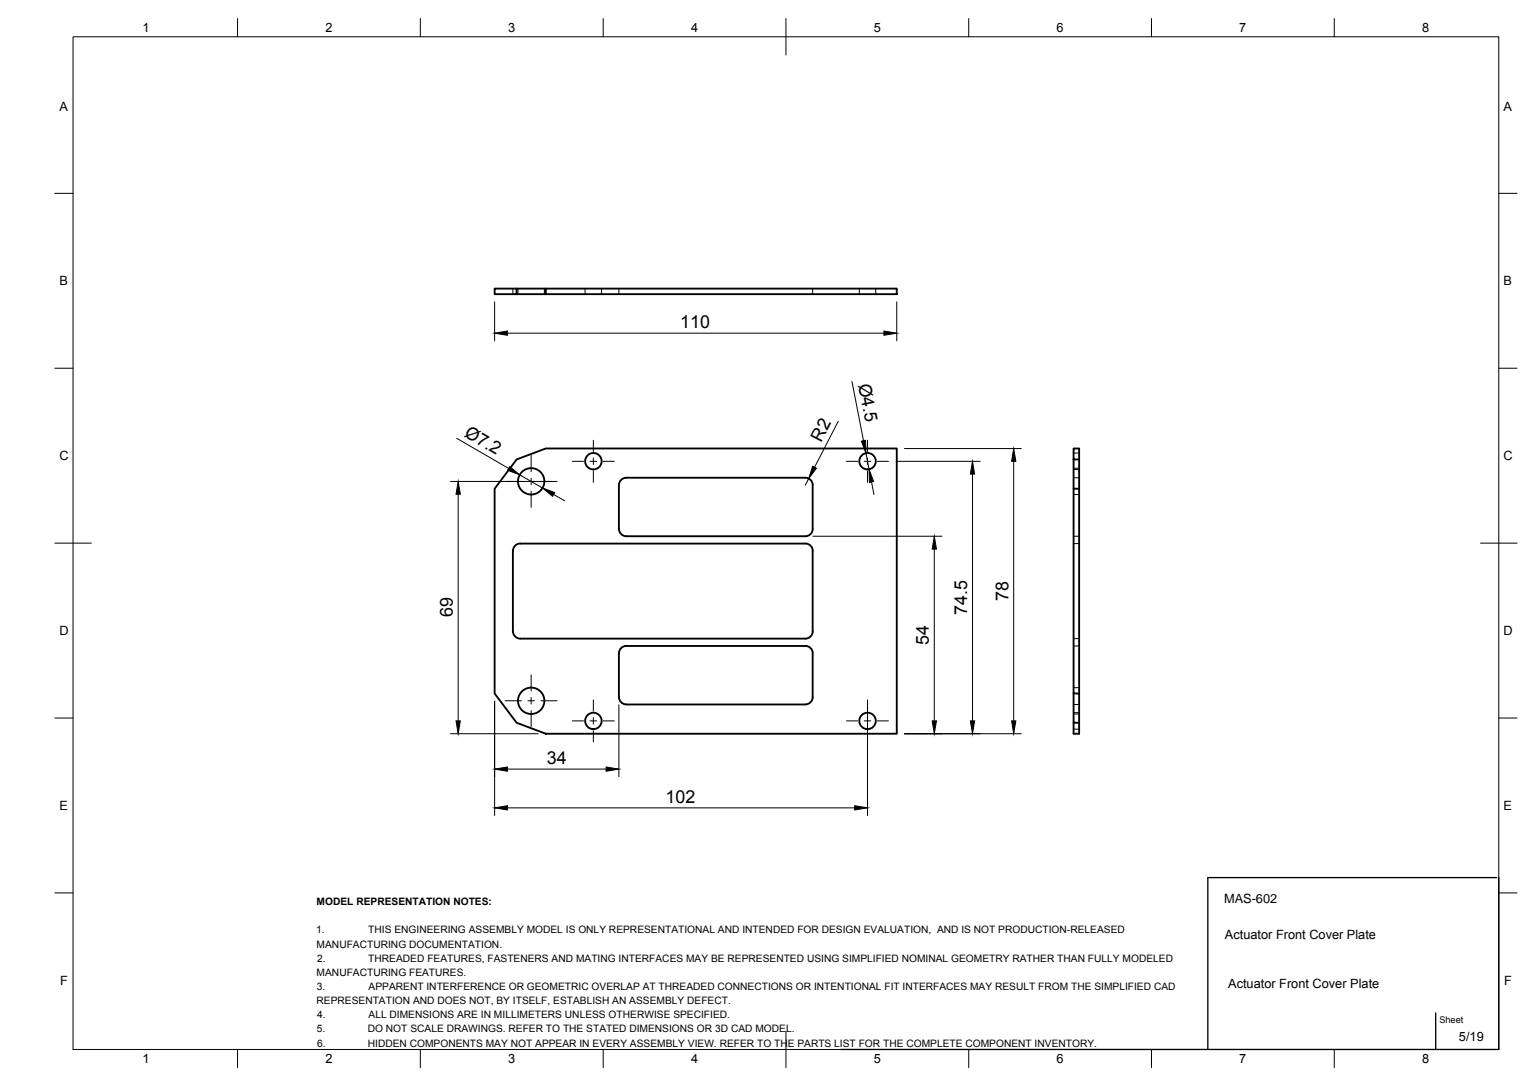
ISO-10303-21;
HEADER;
/* Generated by software containing ST-Developer
 * from STEP Tools, Inc. (www.steptools.com) 
 */

FILE_DESCRIPTION(
/* description */ (''),
/* implementation_level */ '2;1');

FILE_NAME(
/* name */ 'Actuator Front Cover Plate.step',
/* time_stamp */ '2026-10-15T14:42:47-07:00',
/* author */ (''),
/* organization */ (''),
/* preprocessor_version */ 'ST-DEVELOPER v20.2',
/* originating_system */ 'Autodesk Translation Framework v15.15.0.0',
/* authorisation */ '');

FILE_SCHEMA (('AUTOMOTIVE_DESIGN { 1 0 10303 214 3 1 1 }'));
ENDSEC;

DATA;
#10=MECHANICAL_DESIGN_GEOMETRIC_PRESENTATION_REPRESENTATION('',(#236),#85789);
#200=SHAPE_REPRESENTATION_RELATIONSHIP('SRR','None',#85865,#218);
#218=ADVANCED_BREP_SHAPE_REPRESENTATION('',(#254),#85773);
#236=STYLED_ITEM('',(#85964),#254);
#254=MANIFOLD_SOLID_BREP('Body1',#9883);
#411=FACE_BOUND('',#3173,.T.);
#412=FACE_BOUND('',#3174,.T.);
#413=FACE_BOUND('',#3175,.T.);
#414=FACE_BOUND('',#3176,.T.);
#415=FACE_BOUND('',#3177,.T.);
#416=FACE_BOUND('',#3178,.T.);
#417=FACE_BOUND('',#3179,.T.);
#418=FACE_BOUND('',#3180,.T.);
#419=FACE_BOUND('',#3181,.T.);
#420=FACE_BOUND('',#3183,.T.);
#421=FACE_BOUND('',#3184,.T.);
#422=FACE_BOUND('',#3185,.T.);
#423=FACE_BOUND('',#3186,.T.);
#424=FACE_BOUND('',#3187,.T.);
#425=FACE_BOUND('',#3188,.T.);
#426=FACE_BOUND('',#3189,.T.);
#427=FACE_BOUND('',#3190,.T.);
#428=FACE_BOUND('',#3191,.T.);
#1044=PLANE('',#10380);
#1045=PLANE('',#10384);
#1046=PLANE('',#10388);
#1047=PLANE('',#10392);
#1048=PLANE('',#10396);
#1049=PLANE('',#10400);
#1050=PLANE('',#10404);
#1051=PLANE('',#10408);
#1052=PLANE('',#10412);
#1053=PLANE('',#10416);
#1054=PLANE('',#10420);
#1055=PLANE('',#10424);
#1056=PLANE('',#10443);
#1057=PLANE('',#10444);
#1058=PLANE('',#10445);
#1059=PLANE('',#10446);
#1060=PLANE('',#10447);
#1061=PLANE('',#10448);
#1062=PLANE('',#10449);
#1063=PLANE('',#10450);
#1064=PLANE('',#10451);
#1065=PLANE('',#10452);
#1357=LINE('',#23580,#1893);
#1358=LINE('',#23583,#1894);
#1359=LINE('',#23586,#1895);
#1360=LINE('',#23588,#1896);
#1361=LINE('',#23589,#1897);
#1362=LINE('',#23595,#1898);
#1363=LINE('',#23598,#1899);
#1364=LINE('',#23600,#1900);
#1365=LINE('',#23601,#1901);
#1366=LINE('',#23606,#1902);
#1367=LINE('',#23610,#1903);
#1368=LINE('',#23612,#1904);
#1369=LINE('',#23613,#1905);
#1370=LINE('',#23618,#1906);
#1371=LINE('',#23621,#1907);
#1372=LINE('',#23622,#1908);
#1373=LINE('',#23628,#1909);
#1374=LINE('',#23631,#1910);
#1375=LINE('',#23634,#1911);
#1376=LINE('',#23636,#1912);
#1377=LINE('',#23637,#1913);
#1378=LINE('',#23643,#1914);
#1379=LINE('',#23646,#1915);
#1380=LINE('',#23648,#1916);
#1381=LINE('',#23649,#1917);
#1382=LINE('',#23654,#1918);
#1383=LINE('',#23658,#1919);
#1384=LINE('',#23660,#1920);
#1385=LINE('',#23661,#1921);
#1386=LINE('',#23666,#1922);
#1387=LINE('',#23669,#1923);
#1388=LINE('',#23670,#1924);
#1389=LINE('',#23676,#1925);
#1390=LINE('',#23679,#1926);
#1391=LINE('',#23682,#1927);
#1392=LINE('',#23684,#1928);
#1393=LINE('',#23685,#1929);
#1394=LINE('',#23691,#1930);
#1395=LINE('',#23694,#1931);
#1396=LINE('',#23696,#1932);
#1397=LINE('',#23697,#1933);
#1398=LINE('',#23702,#1934);
#1399=LINE('',#23706,#1935);
#1400=LINE('',#23708,#1936);
#1401=LINE('',#23709,#1937);
#1402=LINE('',#23714,#1938);
#1403=LINE('',#23717,#1939);
#1404=LINE('',#23718,#1940);
#1405=LINE('',#23723,#1941);
#1406=LINE('',#23729,#1942);
#1407=LINE('',#23735,#1943);
#1408=LINE('',#23741,#1944);
#1409=LINE('',#23747,#1945);
#1410=LINE('',#23753,#1946);
#1411=LINE('',#23758,#1947);
#1412=LINE('',#23760,#1948);
#1413=LINE('',#23762,#1949);
#1414=LINE('',#23763,#1950);
#1415=LINE('',#23766,#1951);
#1416=LINE('',#23768,#1952);
#1417=LINE('',#23769,#1953);
#1418=LINE('',#23772,#1954);
#1419=LINE('',#23774,#1955);
#1420=LINE('',#23775,#1956);
#1421=LINE('',#23778,#1957);
#1422=LINE('',#23780,#1958);
#1423=LINE('',#23781,#1959);
#1424=LINE('',#23784,#1960);
#1425=LINE('',#23786,#1961);
#1426=LINE('',#23787,#1962);
#1427=LINE('',#23790,#1963);
#1428=LINE('',#23792,#1964);
#1429=LINE('',#23793,#1965);
#1430=LINE('',#23796,#1966);
#1431=LINE('',#23798,#1967);
#1432=LINE('',#23799,#1968);
#1433=LINE('',#23801,#1969);
#1434=LINE('',#23802,#1970);
#1893=VECTOR('',#11679,1.);
#1894=VECTOR('',#11682,1.);
#1895=VECTOR('',#11685,1.);
#1896=VECTOR('',#11686,1.);
#1897=VECTOR('',#11687,1.);
#1898=VECTOR('',#11692,1.);
#1899=VECTOR('',#11695,1.);
#1900=VECTOR('',#11698,1.);
#1901=VECTOR('',#11699,1.);
#1902=VECTOR('',#11704,1.);
#1903=VECTOR('',#11709,1.);
#1904=VECTOR('',#11710,1.);
#1905=VECTOR('',#11711,1.);
#1906=VECTOR('',#11716,1.);
#1907=VECTOR('',#11721,1.);
#1908=VECTOR('',#11722,1.);
#1909=VECTOR('',#11727,1.);
#1910=VECTOR('',#11730,1.);
#1911=VECTOR('',#11733,1.);
#1912=VECTOR('',#11734,1.);
#1913=VECTOR('',#11735,1.);
#1914=VECTOR('',#11740,1.);
#1915=VECTOR('',#11743,1.);
#1916=VECTOR('',#11746,1.);
#1917=VECTOR('',#11747,1.);
#1918=VECTOR('',#11752,1.);
#1919=VECTOR('',#11757,1.);
#1920=VECTOR('',#11758,1.);
#1921=VECTOR('',#11759,1.);
#1922=VECTOR('',#11764,1.);
#1923=VECTOR('',#11769,1.);
#1924=VECTOR('',#11770,1.);
#1925=VECTOR('',#11775,1.);
#1926=VECTOR('',#11778,1.);
#1927=VECTOR('',#11781,1.);
#1928=VECTOR('',#11782,1.);
#1929=VECTOR('',#11783,1.);
#1930=VECTOR('',#11788,1.);
#1931=VECTOR('',#11791,1.);
#1932=VECTOR('',#11794,1.);
#1933=VECTOR('',#11795,1.);
#1934=VECTOR('',#11800,1.);
#1935=VECTOR('',#11805,1.);
#1936=VECTOR('',#11806,1.);
#1937=VECTOR('',#11807,1.);
#1938=VECTOR('',#11812,1.);
#1939=VECTOR('',#11817,1.);
#1940=VECTOR('',#11818,1.);
#1941=VECTOR('',#11823,0.225);
#1942=VECTOR('',#11830,0.36);
#1943=VECTOR('',#11837,0.36);
#1944=VECTOR('',#11844,0.225);
#1945=VECTOR('',#11851,0.225);
#1946=VECTOR('',#11858,0.225);
#1947=VECTOR('',#11863,1.);
#1948=VECTOR('',#11864,1.);
#1949=VECTOR('',#11865,1.);
#1950=VECTOR('',#11866,1.);
#1951=VECTOR('',#11869,1.);
#1952=VECTOR('',#11870,1.);
#1953=VECTOR('',#11871,1.);
#1954=VECTOR('',#11874,1.);
#1955=VECTOR('',#11875,1.);
#1956=VECTOR('',#11876,1.);
#1957=VECTOR('',#11879,1.);
#1958=VECTOR('',#11880,1.);
#1959=VECTOR('',#11881,1.);
#1960=VECTOR('',#11884,1.);
#1961=VECTOR('',#11885,1.);
#1962=VECTOR('',#11886,1.);
#1963=VECTOR('',#11889,1.);
#1964=VECTOR('',#11890,1.);
#1965=VECTOR('',#11891,1.);
#1966=VECTOR('',#11894,1.);
#1967=VECTOR('',#11895,1.);
#1968=VECTOR('',#11896,1.);
#1969=VECTOR('',#11899,1.);
#1970=VECTOR('',#11900,1.);
#2304=CYLINDRICAL_SURFACE('',#10377,0.2);
#2305=CYLINDRICAL_SURFACE('',#10381,0.2);
#2306=CYLINDRICAL_SURFACE('',#10385,0.2);
#2307=CYLINDRICAL_SURFACE('',#10389,0.2);
#2308=CYLINDRICAL_SURFACE('',#10393,0.2);
#2309=CYLINDRICAL_SURFACE('',#10397,0.2);
#2310=CYLINDRICAL_SURFACE('',#10401,0.2);
#2311=CYLINDRICAL_SURFACE('',#10405,0.2);
#2312=CYLINDRICAL_SURFACE('',#10409,0.2);
#2313=CYLINDRICAL_SURFACE('',#10413,0.2);
#2314=CYLINDRICAL_SURFACE('',#10417,0.2);
#2315=CYLINDRICAL_SURFACE('',#10421,0.2);
#2316=CYLINDRICAL_SURFACE('',#10425,0.225);
#2317=CYLINDRICAL_SURFACE('',#10428,0.36);
#2318=CYLINDRICAL_SURFACE('',#10431,0.36);
#2319=CYLINDRICAL_SURFACE('',#10434,0.225);
#2320=CYLINDRICAL_SURFACE('',#10437,0.225);
#2321=CYLINDRICAL_SURFACE('',#10440,0.225);
#2608=FACE_OUTER_BOUND('',#3134,.T.);
#2609=FACE_OUTER_BOUND('',#3135,.T.);
#2610=FACE_OUTER_BOUND('',#3136,.T.);
#2611=FACE_OUTER_BOUND('',#3137,.T.);
#2612=FACE_OUTER_BOUND('',#3138,.T.);
#2613=FACE_OUTER_BOUND('',#3139,.T.);
#2614=FACE_OUTER_BOUND('',#3140,.T.);
#2615=FACE_OUTER_BOUND('',#3141,.T.);
#2616=FACE_OUTER_BOUND('',#3142,.T.);
#2617=FACE_OUTER_BOUND('',#3143,.T.);
#2618=FACE_OUTER_BOUND('',#3144,.T.);
#2619=FACE_OUTER_BOUND('',#3145,.T.);
#2620=FACE_OUTER_BOUND('',#3146,.T.);
#2621=FACE_OUTER_BOUND('',#3147,.T.);
#2622=FACE_OUTER_BOUND('',#3148,.T.);
#2623=FACE_OUTER_BOUND('',#3149,.T.);
#2624=FACE_OUTER_BOUND('',#3150,.T.);
#2625=FACE_OUTER_BOUND('',#3151,.T.);
#2626=FACE_OUTER_BOUND('',#3152,.T.);
#2627=FACE_OUTER_BOUND('',#3153,.T.);
#2628=FACE_OUTER_BOUND('',#3154,.T.);
#2629=FACE_OUTER_BOUND('',#3155,.T.);
#2630=FACE_OUTER_BOUND('',#3156,.T.);
#2631=FACE_OUTER_BOUND('',#3157,.T.);
#2632=FACE_OUTER_BOUND('',#3158,.T.);
#2633=FACE_OUTER_BOUND('',#3159,.T.);
#2634=FACE_OUTER_BOUND('',#3160,.T.);
#2635=FACE_OUTER_BOUND('',#3161,.T.);
#2636=FACE_OUTER_BOUND('',#3162,.T.);
#2637=FACE_OUTER_BOUND('',#3163,.T.);
#2638=FACE_OUTER_BOUND('',#3164,.T.);
#2639=FACE_OUTER_BOUND('',#3165,.T.);
#2640=FACE_OUTER_BOUND('',#3166,.T.);
#2641=FACE_OUTER_BOUND('',#3167,.T.);
#2642=FACE_OUTER_BOUND('',#3168,.T.);
#2643=FACE_OUTER_BOUND('',#3169,.T.);
#2644=FACE_OUTER_BOUND('',#3170,.T.);
#2645=FACE_OUTER_BOUND('',#3171,.T.);
#2646=FACE_OUTER_BOUND('',#3172,.T.);
#2647=FACE_OUTER_BOUND('',#3182,.T.);
#3134=EDGE_LOOP('',(#7413,#7414,#7415,#7416));
#3135=EDGE_LOOP('',(#7417,#7418,#7419,#7420));
#3136=EDGE_LOOP('',(#7421,#7422,#7423,#7424));
#3137=EDGE_LOOP('',(#7425,#7426,#7427,#7428));
#3138=EDGE_LOOP('',(#7429,#7430,#7431,#7432));
#3139=EDGE_LOOP('',(#7433,#7434,#7435,#7436));
#3140=EDGE_LOOP('',(#7437,#7438,#7439,#7440));
#3141=EDGE_LOOP('',(#7441,#7442,#7443,#7444));
#3142=EDGE_LOOP('',(#7445,#7446,#7447,#7448));
#3143=EDGE_LOOP('',(#7449,#7450,#7451,#7452));
#3144=EDGE_LOOP('',(#7453,#7454,#7455,#7456));
#3145=EDGE_LOOP('',(#7457,#7458,#7459,#7460));
#3146=EDGE_LOOP('',(#7461,#7462,#7463,#7464));
#3147=EDGE_LOOP('',(#7465,#7466,#7467,#7468));
#3148=EDGE_LOOP('',(#7469,#7470,#7471,#7472));
#3149=EDGE_LOOP('',(#7473,#7474,#7475,#7476));
#3150=EDGE_LOOP('',(#7477,#7478,#7479,#7480));
#3151=EDGE_LOOP('',(#7481,#7482,#7483,#7484));
#3152=EDGE_LOOP('',(#7485,#7486,#7487,#7488));
#3153=EDGE_LOOP('',(#7489,#7490,#7491,#7492));
#3154=EDGE_LOOP('',(#7493,#7494,#7495,#7496));
#3155=EDGE_LOOP('',(#7497,#7498,#7499,#7500));
#3156=EDGE_LOOP('',(#7501,#7502,#7503,#7504));
#3157=EDGE_LOOP('',(#7505,#7506,#7507,#7508));
#3158=EDGE_LOOP('',(#7509,#7510,#7511,#7512));
#3159=EDGE_LOOP('',(#7513,#7514,#7515,#7516));
#3160=EDGE_LOOP('',(#7517,#7518,#7519,#7520));
#3161=EDGE_LOOP('',(#7521,#7522,#7523,#7524));
#3162=EDGE_LOOP('',(#7525,#7526,#7527,#7528));
#3163=EDGE_LOOP('',(#7529,#7530,#7531,#7532));
#3164=EDGE_LOOP('',(#7533,#7534,#7535,#7536));
#3165=EDGE_LOOP('',(#7537,#7538,#7539,#7540));
#3166=EDGE_LOOP('',(#7541,#7542,#7543,#7544));
#3167=EDGE_LOOP('',(#7545,#7546,#7547,#7548));
#3168=EDGE_LOOP('',(#7549,#7550,#7551,#7552));
#3169=EDGE_LOOP('',(#7553,#7554,#7555,#7556));
#3170=EDGE_LOOP('',(#7557,#7558,#7559,#7560));
#3171=EDGE_LOOP('',(#7561,#7562,#7563,#7564));
#3172=EDGE_LOOP('',(#7565,#7566,#7567,#7568,#7569,#7570,#7571,#7572));
#3173=EDGE_LOOP('',(#7573));
#3174=EDGE_LOOP('',(#7574));
#3175=EDGE_LOOP('',(#7575));
#3176=EDGE_LOOP('',(#7576));
#3177=EDGE_LOOP('',(#7577));
#3178=EDGE_LOOP('',(#7578));
#3179=EDGE_LOOP('',(#7579,#7580,#7581,#7582,#7583,#7584,#7585,#7586));
#3180=EDGE_LOOP('',(#7587,#7588,#7589,#7590,#7591,#7592,#7593,#7594));
#3181=EDGE_LOOP('',(#7595,#7596,#7597,#7598,#7599,#7600,#7601,#7602));
#3182=EDGE_LOOP('',(#7603,#7604,#7605,#7606,#7607,#7608,#7609,#7610));
#3183=EDGE_LOOP('',(#7611));
#3184=EDGE_LOOP('',(#7612));
#3185=EDGE_LOOP('',(#7613));
#3186=EDGE_LOOP('',(#7614));
#3187=EDGE_LOOP('',(#7615));
#3188=EDGE_LOOP('',(#7616));
#3189=EDGE_LOOP('',(#7617,#7618,#7619,#7620,#7621,#7622,#7623,#7624));
#3190=EDGE_LOOP('',(#7625,#7626,#7627,#7628,#7629,#7630,#7631,#7632));
#3191=EDGE_LOOP('',(#7633,#7634,#7635,#7636,#7637,#7638,#7639,#7640));
#3648=CIRCLE('',#10378,0.2);
#3649=CIRCLE('',#10379,0.2);
#3650=CIRCLE('',#10382,0.2);
#3651=CIRCLE('',#10383,0.2);
#3652=CIRCLE('',#10386,0.2);
#3653=CIRCLE('',#10387,0.2);
#3654=CIRCLE('',#10390,0.2);
#3655=CIRCLE('',#10391,0.2);
#3656=CIRCLE('',#10394,0.2);
#3657=CIRCLE('',#10395,0.2);
#3658=CIRCLE('',#10398,0.2);
#3659=CIRCLE('',#10399,0.2);
#3660=CIRCLE('',#10402,0.2);
#3661=CIRCLE('',#10403,0.2);
#3662=CIRCLE('',#10406,0.2);
#3663=CIRCLE('',#10407,0.2);
#3664=CIRCLE('',#10410,0.2);
#3665=CIRCLE('',#10411,0.2);
#3666=CIRCLE('',#10414,0.2);
#3667=CIRCLE('',#10415,0.2);
#3668=CIRCLE('',#10418,0.2);
#3669=CIRCLE('',#10419,0.2);
#3670=CIRCLE('',#10422,0.2);
#3671=CIRCLE('',#10423,0.2);
#3672=CIRCLE('',#10426,0.225);
#3673=CIRCLE('',#10427,0.225);
#3674=CIRCLE('',#10429,0.36);
#3675=CIRCLE('',#10430,0.36);
#3676=CIRCLE('',#10432,0.36);
#3677=CIRCLE('',#10433,0.36);
#3678=CIRCLE('',#10435,0.225);
#3679=CIRCLE('',#10436,0.225);
#3680=CIRCLE('',#10438,0.225);
#3681=CIRCLE('',#10439,0.225);
#3682=CIRCLE('',#10441,0.225);
#3683=CIRCLE('',#10442,0.225);
#4199=VERTEX_POINT('',#23576);
#4200=VERTEX_POINT('',#23577);
#4201=VERTEX_POINT('',#23579);
#4202=VERTEX_POINT('',#23581);
#4203=VERTEX_POINT('',#23585);
#4204=VERTEX_POINT('',#23587);
#4205=VERTEX_POINT('',#23591);
#4206=VERTEX_POINT('',#23592);
#4207=VERTEX_POINT('',#23594);
#4208=VERTEX_POINT('',#23596);
#4209=VERTEX_POINT('',#23603);
#4210=VERTEX_POINT('',#23605);
#4211=VERTEX_POINT('',#23609);
#4212=VERTEX_POINT('',#23611);
#4213=VERTEX_POINT('',#23615);
#4214=VERTEX_POINT('',#23617);
#4215=VERTEX_POINT('',#23624);
#4216=VERTEX_POINT('',#23625);
#4217=VERTEX_POINT('',#23627);
#4218=VERTEX_POINT('',#23629);
#4219=VERTEX_POINT('',#23633);
#4220=VERTEX_POINT('',#23635);
#4221=VERTEX_POINT('',#23639);
#4222=VERTEX_POINT('',#23640);
#4223=VERTEX_POINT('',#23642);
#4224=VERTEX_POINT('',#23644);
#4225=VERTEX_POINT('',#23651);
#4226=VERTEX_POINT('',#23653);
#4227=VERTEX_POINT('',#23657);
#4228=VERTEX_POINT('',#23659);
#4229=VERTEX_POINT('',#23663);
#4230=VERTEX_POINT('',#23665);
#4231=VERTEX_POINT('',#23672);
#4232=VERTEX_POINT('',#23673);
#4233=VERTEX_POINT('',#23675);
#4234=VERTEX_POINT('',#23677);
#4235=VERTEX_POINT('',#23681);
#4236=VERTEX_POINT('',#23683);
#4237=VERTEX_POINT('',#23687);
#4238=VERTEX_POINT('',#23688);
#4239=VERTEX_POINT('',#23690);
#4240=VERTEX_POINT('',#23692);
#4241=VERTEX_POINT('',#23699);
#4242=VERTEX_POINT('',#23701);
#4243=VERTEX_POINT('',#23705);
#4244=VERTEX_POINT('',#23707);
#4245=VERTEX_POINT('',#23711);
#4246=VERTEX_POINT('',#23713);
#4247=VERTEX_POINT('',#23720);
#4248=VERTEX_POINT('',#23722);
#4249=VERTEX_POINT('',#23726);
#4250=VERTEX_POINT('',#23728);
#4251=VERTEX_POINT('',#23732);
#4252=VERTEX_POINT('',#23734);
#4253=VERTEX_POINT('',#23738);
#4254=VERTEX_POINT('',#23740);
#4255=VERTEX_POINT('',#23744);
#4256=VERTEX_POINT('',#23746);
#4257=VERTEX_POINT('',#23750);
#4258=VERTEX_POINT('',#23752);
#4259=VERTEX_POINT('',#23756);
#4260=VERTEX_POINT('',#23757);
#4261=VERTEX_POINT('',#23759);
#4262=VERTEX_POINT('',#23761);
#4263=VERTEX_POINT('',#23765);
#4264=VERTEX_POINT('',#23767);
#4265=VERTEX_POINT('',#23771);
#4266=VERTEX_POINT('',#23773);
#4267=VERTEX_POINT('',#23777);
#4268=VERTEX_POINT('',#23779);
#4269=VERTEX_POINT('',#23783);
#4270=VERTEX_POINT('',#23785);
#4271=VERTEX_POINT('',#23789);
#4272=VERTEX_POINT('',#23791);
#4273=VERTEX_POINT('',#23795);
#4274=VERTEX_POINT('',#23797);
#5434=EDGE_CURVE('',#4199,#4200,#3648,.T.);
#5435=EDGE_CURVE('',#4200,#4201,#1357,.T.);
#5436=EDGE_CURVE('',#4201,#4202,#3649,.T.);
#5437=EDGE_CURVE('',#4202,#4199,#1358,.T.);
#5438=EDGE_CURVE('',#4203,#4200,#1359,.T.);
#5439=EDGE_CURVE('',#4204,#4203,#1360,.T.);
#5440=EDGE_CURVE('',#4201,#4204,#1361,.T.);
#5441=EDGE_CURVE('',#4205,#4206,#3650,.T.);
#5442=EDGE_CURVE('',#4206,#4207,#1362,.T.);
#5443=EDGE_CURVE('',#4207,#4208,#3651,.T.);
#5444=EDGE_CURVE('',#4208,#4205,#1363,.T.);
#5445=EDGE_CURVE('',#4207,#4202,#1364,.T.);
#5446=EDGE_CURVE('',#4199,#4206,#1365,.T.);
#5447=EDGE_CURVE('',#4203,#4209,#3652,.T.);
#5448=EDGE_CURVE('',#4209,#4210,#1366,.T.);
#5449=EDGE_CURVE('',#4210,#4204,#3653,.T.);
#5450=EDGE_CURVE('',#4211,#4209,#1367,.T.);
#5451=EDGE_CURVE('',#4212,#4211,#1368,.T.);
#5452=EDGE_CURVE('',#4210,#4212,#1369,.T.);
#5453=EDGE_CURVE('',#4211,#4213,#3654,.T.);
#5454=EDGE_CURVE('',#4213,#4214,#1370,.T.);
#5455=EDGE_CURVE('',#4214,#4212,#3655,.T.);
#5456=EDGE_CURVE('',#4214,#4208,#1371,.T.);
#5457=EDGE_CURVE('',#4205,#4213,#1372,.T.);
#5458=EDGE_CURVE('',#4215,#4216,#3656,.T.);
#5459=EDGE_CURVE('',#4216,#4217,#1373,.T.);
#5460=EDGE_CURVE('',#4217,#4218,#3657,.T.);
#5461=EDGE_CURVE('',#4218,#4215,#1374,.T.);
#5462=EDGE_CURVE('',#4219,#4216,#1375,.T.);
#5463=EDGE_CURVE('',#4220,#4219,#1376,.T.);
#5464=EDGE_CURVE('',#4217,#4220,#1377,.T.);
#5465=EDGE_CURVE('',#4221,#4222,#3658,.T.);
#5466=EDGE_CURVE('',#4222,#4223,#1378,.T.);
#5467=EDGE_CURVE('',#4223,#4224,#3659,.T.);
#5468=EDGE_CURVE('',#4224,#4221,#1379,.T.);
#5469=EDGE_CURVE('',#4223,#4218,#1380,.T.);
#5470=EDGE_CURVE('',#4215,#4222,#1381,.T.);
#5471=EDGE_CURVE('',#4219,#4225,#3660,.T.);
#5472=EDGE_CURVE('',#4225,#4226,#1382,.T.);
#5473=EDGE_CURVE('',#4226,#4220,#3661,.T.);
#5474=EDGE_CURVE('',#4227,#4225,#1383,.T.);
#5475=EDGE_CURVE('',#4228,#4227,#1384,.T.);
#5476=EDGE_CURVE('',#4226,#4228,#1385,.T.);
#5477=EDGE_CURVE('',#4227,#4229,#3662,.T.);
#5478=EDGE_CURVE('',#4229,#4230,#1386,.T.);
#5479=EDGE_CURVE('',#4230,#4228,#3663,.T.);
#5480=EDGE_CURVE('',#4230,#4224,#1387,.T.);
#5481=EDGE_CURVE('',#4221,#4229,#1388,.T.);
#5482=EDGE_CURVE('',#4231,#4232,#3664,.T.);
#5483=EDGE_CURVE('',#4232,#4233,#1389,.T.);
#5484=EDGE_CURVE('',#4233,#4234,#3665,.T.);
#5485=EDGE_CURVE('',#4234,#4231,#1390,.T.);
#5486=EDGE_CURVE('',#4235,#4232,#1391,.T.);
#5487=EDGE_CURVE('',#4236,#4235,#1392,.T.);
#5488=EDGE_CURVE('',#4233,#4236,#1393,.T.);
#5489=EDGE_CURVE('',#4237,#4238,#3666,.T.);
#5490=EDGE_CURVE('',#4238,#4239,#1394,.T.);
#5491=EDGE_CURVE('',#4239,#4240,#3667,.T.);
#5492=EDGE_CURVE('',#4240,#4237,#1395,.T.);
#5493=EDGE_CURVE('',#4239,#4234,#1396,.T.);
#5494=EDGE_CURVE('',#4231,#4238,#1397,.T.);
#5495=EDGE_CURVE('',#4235,#4241,#3668,.T.);
#5496=EDGE_CURVE('',#4241,#4242,#1398,.T.);
#5497=EDGE_CURVE('',#4242,#4236,#3669,.T.);
#5498=EDGE_CURVE('',#4243,#4241,#1399,.T.);
#5499=EDGE_CURVE('',#4244,#4243,#1400,.T.);
#5500=EDGE_CURVE('',#4242,#4244,#1401,.T.);
#5501=EDGE_CURVE('',#4243,#4245,#3670,.T.);
#5502=EDGE_CURVE('',#4245,#4246,#1402,.T.);
#5503=EDGE_CURVE('',#4246,#4244,#3671,.T.);
#5504=EDGE_CURVE('',#4246,#4240,#1403,.T.);
#5505=EDGE_CURVE('',#4237,#4245,#1404,.T.);
#5506=EDGE_CURVE('',#4247,#4247,#3672,.T.);
#5507=EDGE_CURVE('',#4247,#4248,#1405,.T.);
#5508=EDGE_CURVE('',#4248,#4248,#3673,.T.);
#5509=EDGE_CURVE('',#4249,#4249,#3674,.T.);
#5510=EDGE_CURVE('',#4249,#4250,#1406,.T.);
#5511=EDGE_CURVE('',#4250,#4250,#3675,.T.);
#5512=EDGE_CURVE('',#4251,#4251,#3676,.T.);
#5513=EDGE_CURVE('',#4251,#4252,#1407,.T.);
#5514=EDGE_CURVE('',#4252,#4252,#3677,.T.);
#5515=EDGE_CURVE('',#4253,#4253,#3678,.T.);
#5516=EDGE_CURVE('',#4253,#4254,#1408,.T.);
#5517=EDGE_CURVE('',#4254,#4254,#3679,.T.);
#5518=EDGE_CURVE('',#4255,#4255,#3680,.T.);
#5519=EDGE_CURVE('',#4255,#4256,#1409,.T.);
#5520=EDGE_CURVE('',#4256,#4256,#3681,.T.);
#5521=EDGE_CURVE('',#4257,#4257,#3682,.T.);
#5522=EDGE_CURVE('',#4257,#4258,#1410,.T.);
#5523=EDGE_CURVE('',#4258,#4258,#3683,.T.);
#5524=EDGE_CURVE('',#4259,#4260,#1411,.T.);
#5525=EDGE_CURVE('',#4259,#4261,#1412,.T.);
#5526=EDGE_CURVE('',#4262,#4261,#1413,.T.);
#5527=EDGE_CURVE('',#4260,#4262,#1414,.T.);
#5528=EDGE_CURVE('',#4260,#4263,#1415,.T.);
#5529=EDGE_CURVE('',#4264,#4262,#1416,.T.);
#5530=EDGE_CURVE('',#4263,#4264,#1417,.T.);
#5531=EDGE_CURVE('',#4263,#4265,#1418,.T.);
#5532=EDGE_CURVE('',#4266,#4264,#1419,.T.);
#5533=EDGE_CURVE('',#4265,#4266,#1420,.T.);
#5534=EDGE_CURVE('',#4265,#4267,#1421,.T.);
#5535=EDGE_CURVE('',#4268,#4266,#1422,.T.);
#5536=EDGE_CURVE('',#4267,#4268,#1423,.T.);
#5537=EDGE_CURVE('',#4267,#4269,#1424,.T.);
#5538=EDGE_CURVE('',#4270,#4268,#1425,.T.);
#5539=EDGE_CURVE('',#4269,#4270,#1426,.T.);
#5540=EDGE_CURVE('',#4269,#4271,#1427,.T.);
#5541=EDGE_CURVE('',#4272,#4270,#1428,.T.);
#5542=EDGE_CURVE('',#4271,#4272,#1429,.T.);
#5543=EDGE_CURVE('',#4271,#4273,#1430,.T.);
#5544=EDGE_CURVE('',#4274,#4272,#1431,.T.);
#5545=EDGE_CURVE('',#4273,#4274,#1432,.T.);
#5546=EDGE_CURVE('',#4273,#4259,#1433,.T.);
#5547=EDGE_CURVE('',#4261,#4274,#1434,.T.);
#7413=ORIENTED_EDGE('',*,*,#5434,.T.);
#7414=ORIENTED_EDGE('',*,*,#5435,.T.);
#7415=ORIENTED_EDGE('',*,*,#5436,.T.);
#7416=ORIENTED_EDGE('',*,*,#5437,.T.);
#7417=ORIENTED_EDGE('',*,*,#5435,.F.);
#7418=ORIENTED_EDGE('',*,*,#5438,.F.);
#7419=ORIENTED_EDGE('',*,*,#5439,.F.);
#7420=ORIENTED_EDGE('',*,*,#5440,.F.);
#7421=ORIENTED_EDGE('',*,*,#5441,.T.);
#7422=ORIENTED_EDGE('',*,*,#5442,.T.);
#7423=ORIENTED_EDGE('',*,*,#5443,.T.);
#7424=ORIENTED_EDGE('',*,*,#5444,.T.);
#7425=ORIENTED_EDGE('',*,*,#5437,.F.);
#7426=ORIENTED_EDGE('',*,*,#5445,.F.);
#7427=ORIENTED_EDGE('',*,*,#5442,.F.);
#7428=ORIENTED_EDGE('',*,*,#5446,.F.);
#7429=ORIENTED_EDGE('',*,*,#5447,.T.);
#7430=ORIENTED_EDGE('',*,*,#5448,.T.);
#7431=ORIENTED_EDGE('',*,*,#5449,.T.);
#7432=ORIENTED_EDGE('',*,*,#5439,.T.);
#7433=ORIENTED_EDGE('',*,*,#5448,.F.);
#7434=ORIENTED_EDGE('',*,*,#5450,.F.);
#7435=ORIENTED_EDGE('',*,*,#5451,.F.);
#7436=ORIENTED_EDGE('',*,*,#5452,.F.);
#7437=ORIENTED_EDGE('',*,*,#5453,.T.);
#7438=ORIENTED_EDGE('',*,*,#5454,.T.);
#7439=ORIENTED_EDGE('',*,*,#5455,.T.);
#7440=ORIENTED_EDGE('',*,*,#5451,.T.);
#7441=ORIENTED_EDGE('',*,*,#5444,.F.);
#7442=ORIENTED_EDGE('',*,*,#5456,.F.);
#7443=ORIENTED_EDGE('',*,*,#5454,.F.);
#7444=ORIENTED_EDGE('',*,*,#5457,.F.);
#7445=ORIENTED_EDGE('',*,*,#5458,.T.);
#7446=ORIENTED_EDGE('',*,*,#5459,.T.);
#7447=ORIENTED_EDGE('',*,*,#5460,.T.);
#7448=ORIENTED_EDGE('',*,*,#5461,.T.);
#7449=ORIENTED_EDGE('',*,*,#5459,.F.);
#7450=ORIENTED_EDGE('',*,*,#5462,.F.);
#7451=ORIENTED_EDGE('',*,*,#5463,.F.);
#7452=ORIENTED_EDGE('',*,*,#5464,.F.);
#7453=ORIENTED_EDGE('',*,*,#5465,.T.);
#7454=ORIENTED_EDGE('',*,*,#5466,.T.);
#7455=ORIENTED_EDGE('',*,*,#5467,.T.);
#7456=ORIENTED_EDGE('',*,*,#5468,.T.);
#7457=ORIENTED_EDGE('',*,*,#5461,.F.);
#7458=ORIENTED_EDGE('',*,*,#5469,.F.);
#7459=ORIENTED_EDGE('',*,*,#5466,.F.);
#7460=ORIENTED_EDGE('',*,*,#5470,.F.);
#7461=ORIENTED_EDGE('',*,*,#5471,.T.);
#7462=ORIENTED_EDGE('',*,*,#5472,.T.);
#7463=ORIENTED_EDGE('',*,*,#5473,.T.);
#7464=ORIENTED_EDGE('',*,*,#5463,.T.);
#7465=ORIENTED_EDGE('',*,*,#5472,.F.);
#7466=ORIENTED_EDGE('',*,*,#5474,.F.);
#7467=ORIENTED_EDGE('',*,*,#5475,.F.);
#7468=ORIENTED_EDGE('',*,*,#5476,.F.);
#7469=ORIENTED_EDGE('',*,*,#5477,.T.);
#7470=ORIENTED_EDGE('',*,*,#5478,.T.);
#7471=ORIENTED_EDGE('',*,*,#5479,.T.);
#7472=ORIENTED_EDGE('',*,*,#5475,.T.);
#7473=ORIENTED_EDGE('',*,*,#5468,.F.);
#7474=ORIENTED_EDGE('',*,*,#5480,.F.);
#7475=ORIENTED_EDGE('',*,*,#5478,.F.);
#7476=ORIENTED_EDGE('',*,*,#5481,.F.);
#7477=ORIENTED_EDGE('',*,*,#5482,.T.);
#7478=ORIENTED_EDGE('',*,*,#5483,.T.);
#7479=ORIENTED_EDGE('',*,*,#5484,.T.);
#7480=ORIENTED_EDGE('',*,*,#5485,.T.);
#7481=ORIENTED_EDGE('',*,*,#5483,.F.);
#7482=ORIENTED_EDGE('',*,*,#5486,.F.);
#7483=ORIENTED_EDGE('',*,*,#5487,.F.);
#7484=ORIENTED_EDGE('',*,*,#5488,.F.);
#7485=ORIENTED_EDGE('',*,*,#5489,.T.);
#7486=ORIENTED_EDGE('',*,*,#5490,.T.);
#7487=ORIENTED_EDGE('',*,*,#5491,.T.);
#7488=ORIENTED_EDGE('',*,*,#5492,.T.);
#7489=ORIENTED_EDGE('',*,*,#5485,.F.);
#7490=ORIENTED_EDGE('',*,*,#5493,.F.);
#7491=ORIENTED_EDGE('',*,*,#5490,.F.);
#7492=ORIENTED_EDGE('',*,*,#5494,.F.);
#7493=ORIENTED_EDGE('',*,*,#5495,.T.);
#7494=ORIENTED_EDGE('',*,*,#5496,.T.);
#7495=ORIENTED_EDGE('',*,*,#5497,.T.);
#7496=ORIENTED_EDGE('',*,*,#5487,.T.);
#7497=ORIENTED_EDGE('',*,*,#5496,.F.);
#7498=ORIENTED_EDGE('',*,*,#5498,.F.);
#7499=ORIENTED_EDGE('',*,*,#5499,.F.);
#7500=ORIENTED_EDGE('',*,*,#5500,.F.);
#7501=ORIENTED_EDGE('',*,*,#5501,.T.);
#7502=ORIENTED_EDGE('',*,*,#5502,.T.);
#7503=ORIENTED_EDGE('',*,*,#5503,.T.);
#7504=ORIENTED_EDGE('',*,*,#5499,.T.);
#7505=ORIENTED_EDGE('',*,*,#5492,.F.);
#7506=ORIENTED_EDGE('',*,*,#5504,.F.);
#7507=ORIENTED_EDGE('',*,*,#5502,.F.);
#7508=ORIENTED_EDGE('',*,*,#5505,.F.);
#7509=ORIENTED_EDGE('',*,*,#5506,.F.);
#7510=ORIENTED_EDGE('',*,*,#5507,.T.);
#7511=ORIENTED_EDGE('',*,*,#5508,.F.);
#7512=ORIENTED_EDGE('',*,*,#5507,.F.);
#7513=ORIENTED_EDGE('',*,*,#5509,.F.);
#7514=ORIENTED_EDGE('',*,*,#5510,.T.);
#7515=ORIENTED_EDGE('',*,*,#5511,.F.);
#7516=ORIENTED_EDGE('',*,*,#5510,.F.);
#7517=ORIENTED_EDGE('',*,*,#5512,.F.);
#7518=ORIENTED_EDGE('',*,*,#5513,.T.);
#7519=ORIENTED_EDGE('',*,*,#5514,.F.);
#7520=ORIENTED_EDGE('',*,*,#5513,.F.);
#7521=ORIENTED_EDGE('',*,*,#5515,.F.);
#7522=ORIENTED_EDGE('',*,*,#5516,.T.);
#7523=ORIENTED_EDGE('',*,*,#5517,.F.);
#7524=ORIENTED_EDGE('',*,*,#5516,.F.);
#7525=ORIENTED_EDGE('',*,*,#5518,.F.);
#7526=ORIENTED_EDGE('',*,*,#5519,.T.);
#7527=ORIENTED_EDGE('',*,*,#5520,.F.);
#7528=ORIENTED_EDGE('',*,*,#5519,.F.);
#7529=ORIENTED_EDGE('',*,*,#5521,.F.);
#7530=ORIENTED_EDGE('',*,*,#5522,.T.);
#7531=ORIENTED_EDGE('',*,*,#5523,.F.);
#7532=ORIENTED_EDGE('',*,*,#5522,.F.);
#7533=ORIENTED_EDGE('',*,*,#5524,.F.);
#7534=ORIENTED_EDGE('',*,*,#5525,.T.);
#7535=ORIENTED_EDGE('',*,*,#5526,.F.);
#7536=ORIENTED_EDGE('',*,*,#5527,.F.);
#7537=ORIENTED_EDGE('',*,*,#5528,.F.);
#7538=ORIENTED_EDGE('',*,*,#5527,.T.);
#7539=ORIENTED_EDGE('',*,*,#5529,.F.);
#7540=ORIENTED_EDGE('',*,*,#5530,.F.);
#7541=ORIENTED_EDGE('',*,*,#5531,.F.);
#7542=ORIENTED_EDGE('',*,*,#5530,.T.);
#7543=ORIENTED_EDGE('',*,*,#5532,.F.);
#7544=ORIENTED_EDGE('',*,*,#5533,.F.);
#7545=ORIENTED_EDGE('',*,*,#5534,.F.);
#7546=ORIENTED_EDGE('',*,*,#5533,.T.);
#7547=ORIENTED_EDGE('',*,*,#5535,.F.);
#7548=ORIENTED_EDGE('',*,*,#5536,.F.);
#7549=ORIENTED_EDGE('',*,*,#5537,.F.);
#7550=ORIENTED_EDGE('',*,*,#5536,.T.);
#7551=ORIENTED_EDGE('',*,*,#5538,.F.);
#7552=ORIENTED_EDGE('',*,*,#5539,.F.);
#7553=ORIENTED_EDGE('',*,*,#5540,.F.);
#7554=ORIENTED_EDGE('',*,*,#5539,.T.);
#7555=ORIENTED_EDGE('',*,*,#5541,.F.);
#7556=ORIENTED_EDGE('',*,*,#5542,.F.);
#7557=ORIENTED_EDGE('',*,*,#5543,.F.);
#7558=ORIENTED_EDGE('',*,*,#5542,.T.);
#7559=ORIENTED_EDGE('',*,*,#5544,.F.);
#7560=ORIENTED_EDGE('',*,*,#5545,.F.);
#7561=ORIENTED_EDGE('',*,*,#5546,.F.);
#7562=ORIENTED_EDGE('',*,*,#5545,.T.);
#7563=ORIENTED_EDGE('',*,*,#5547,.F.);
#7564=ORIENTED_EDGE('',*,*,#5525,.F.);
#7565=ORIENTED_EDGE('',*,*,#5547,.T.);
#7566=ORIENTED_EDGE('',*,*,#5544,.T.);
#7567=ORIENTED_EDGE('',*,*,#5541,.T.);
#7568=ORIENTED_EDGE('',*,*,#5538,.T.);
#7569=ORIENTED_EDGE('',*,*,#5535,.T.);
#7570=ORIENTED_EDGE('',*,*,#5532,.T.);
#7571=ORIENTED_EDGE('',*,*,#5529,.T.);
#7572=ORIENTED_EDGE('',*,*,#5526,.T.);
#7573=ORIENTED_EDGE('',*,*,#5508,.T.);
#7574=ORIENTED_EDGE('',*,*,#5511,.T.);
#7575=ORIENTED_EDGE('',*,*,#5514,.T.);
#7576=ORIENTED_EDGE('',*,*,#5517,.T.);
#7577=ORIENTED_EDGE('',*,*,#5520,.T.);
#7578=ORIENTED_EDGE('',*,*,#5523,.T.);
#7579=ORIENTED_EDGE('',*,*,#5452,.T.);
#7580=ORIENTED_EDGE('',*,*,#5455,.F.);
#7581=ORIENTED_EDGE('',*,*,#5456,.T.);
#7582=ORIENTED_EDGE('',*,*,#5443,.F.);
#7583=ORIENTED_EDGE('',*,*,#5445,.T.);
#7584=ORIENTED_EDGE('',*,*,#5436,.F.);
#7585=ORIENTED_EDGE('',*,*,#5440,.T.);
#7586=ORIENTED_EDGE('',*,*,#5449,.F.);
#7587=ORIENTED_EDGE('',*,*,#5476,.T.);
#7588=ORIENTED_EDGE('',*,*,#5479,.F.);
#7589=ORIENTED_EDGE('',*,*,#5480,.T.);
#7590=ORIENTED_EDGE('',*,*,#5467,.F.);
#7591=ORIENTED_EDGE('',*,*,#5469,.T.);
#7592=ORIENTED_EDGE('',*,*,#5460,.F.);
#7593=ORIENTED_EDGE('',*,*,#5464,.T.);
#7594=ORIENTED_EDGE('',*,*,#5473,.F.);
#7595=ORIENTED_EDGE('',*,*,#5500,.T.);
#7596=ORIENTED_EDGE('',*,*,#5503,.F.);
#7597=ORIENTED_EDGE('',*,*,#5504,.T.);
#7598=ORIENTED_EDGE('',*,*,#5491,.F.);
#7599=ORIENTED_EDGE('',*,*,#5493,.T.);
#7600=ORIENTED_EDGE('',*,*,#5484,.F.);
#7601=ORIENTED_EDGE('',*,*,#5488,.T.);
#7602=ORIENTED_EDGE('',*,*,#5497,.F.);
#7603=ORIENTED_EDGE('',*,*,#5546,.T.);
#7604=ORIENTED_EDGE('',*,*,#5524,.T.);
#7605=ORIENTED_EDGE('',*,*,#5528,.T.);
#7606=ORIENTED_EDGE('',*,*,#5531,.T.);
#7607=ORIENTED_EDGE('',*,*,#5534,.T.);
#7608=ORIENTED_EDGE('',*,*,#5537,.T.);
#7609=ORIENTED_EDGE('',*,*,#5540,.T.);
#7610=ORIENTED_EDGE('',*,*,#5543,.T.);
#7611=ORIENTED_EDGE('',*,*,#5506,.T.);
#7612=ORIENTED_EDGE('',*,*,#5509,.T.);
#7613=ORIENTED_EDGE('',*,*,#5512,.T.);
#7614=ORIENTED_EDGE('',*,*,#5515,.T.);
#7615=ORIENTED_EDGE('',*,*,#5518,.T.);
#7616=ORIENTED_EDGE('',*,*,#5521,.T.);
#7617=ORIENTED_EDGE('',*,*,#5450,.T.);
#7618=ORIENTED_EDGE('',*,*,#5447,.F.);
#7619=ORIENTED_EDGE('',*,*,#5438,.T.);
#7620=ORIENTED_EDGE('',*,*,#5434,.F.);
#7621=ORIENTED_EDGE('',*,*,#5446,.T.);
#7622=ORIENTED_EDGE('',*,*,#5441,.F.);
#7623=ORIENTED_EDGE('',*,*,#5457,.T.);
#7624=ORIENTED_EDGE('',*,*,#5453,.F.);
#7625=ORIENTED_EDGE('',*,*,#5474,.T.);
#7626=ORIENTED_EDGE('',*,*,#5471,.F.);
#7627=ORIENTED_EDGE('',*,*,#5462,.T.);
#7628=ORIENTED_EDGE('',*,*,#5458,.F.);
#7629=ORIENTED_EDGE('',*,*,#5470,.T.);
#7630=ORIENTED_EDGE('',*,*,#5465,.F.);
#7631=ORIENTED_EDGE('',*,*,#5481,.T.);
#7632=ORIENTED_EDGE('',*,*,#5477,.F.);
#7633=ORIENTED_EDGE('',*,*,#5498,.T.);
#7634=ORIENTED_EDGE('',*,*,#5495,.F.);
#7635=ORIENTED_EDGE('',*,*,#5486,.T.);
#7636=ORIENTED_EDGE('',*,*,#5482,.F.);
#7637=ORIENTED_EDGE('',*,*,#5494,.T.);
#7638=ORIENTED_EDGE('',*,*,#5489,.F.);
#7639=ORIENTED_EDGE('',*,*,#5505,.T.);
#7640=ORIENTED_EDGE('',*,*,#5501,.F.);
#9586=ADVANCED_FACE('',(#2608),#2304,.F.);
#9587=ADVANCED_FACE('',(#2609),#1044,.F.);
#9588=ADVANCED_FACE('',(#2610),#2305,.F.);
#9589=ADVANCED_FACE('',(#2611),#1045,.F.);
#9590=ADVANCED_FACE('',(#2612),#2306,.F.);
#9591=ADVANCED_FACE('',(#2613),#1046,.F.);
#9592=ADVANCED_FACE('',(#2614),#2307,.F.);
#9593=ADVANCED_FACE('',(#2615),#1047,.F.);
#9594=ADVANCED_FACE('',(#2616),#2308,.F.);
#9595=ADVANCED_FACE('',(#2617),#1048,.F.);
#9596=ADVANCED_FACE('',(#2618),#2309,.F.);
#9597=ADVANCED_FACE('',(#2619),#1049,.F.);
#9598=ADVANCED_FACE('',(#2620),#2310,.F.);
#9599=ADVANCED_FACE('',(#2621),#1050,.F.);
#9600=ADVANCED_FACE('',(#2622),#2311,.F.);
#9601=ADVANCED_FACE('',(#2623),#1051,.F.);
#9602=ADVANCED_FACE('',(#2624),#2312,.F.);
#9603=ADVANCED_FACE('',(#2625),#1052,.F.);
#9604=ADVANCED_FACE('',(#2626),#2313,.F.);
#9605=ADVANCED_FACE('',(#2627),#1053,.F.);
#9606=ADVANCED_FACE('',(#2628),#2314,.F.);
#9607=ADVANCED_FACE('',(#2629),#1054,.F.);
#9608=ADVANCED_FACE('',(#2630),#2315,.F.);
#9609=ADVANCED_FACE('',(#2631),#1055,.F.);
#9610=ADVANCED_FACE('',(#2632),#2316,.F.);
#9611=ADVANCED_FACE('',(#2633),#2317,.F.);
#9612=ADVANCED_FACE('',(#2634),#2318,.F.);
#9613=ADVANCED_FACE('',(#2635),#2319,.F.);
#9614=ADVANCED_FACE('',(#2636),#2320,.F.);
#9615=ADVANCED_FACE('',(#2637),#2321,.F.);
#9616=ADVANCED_FACE('',(#2638),#1056,.T.);
#9617=ADVANCED_FACE('',(#2639),#1057,.T.);
#9618=ADVANCED_FACE('',(#2640),#1058,.T.);
#9619=ADVANCED_FACE('',(#2641),#1059,.T.);
#9620=ADVANCED_FACE('',(#2642),#1060,.T.);
#9621=ADVANCED_FACE('',(#2643),#1061,.T.);
#9622=ADVANCED_FACE('',(#2644),#1062,.T.);
#9623=ADVANCED_FACE('',(#2645),#1063,.T.);
#9624=ADVANCED_FACE('',(#2646,#411,#412,#413,#414,#415,#416,#417,#418,#419),
#1064,.T.);
#9625=ADVANCED_FACE('',(#2647,#420,#421,#422,#423,#424,#425,#426,#427,#428),
#1065,.F.);
#9883=CLOSED_SHELL('',(#9586,#9587,#9588,#9589,#9590,#9591,#9592,#9593,
#9594,#9595,#9596,#9597,#9598,#9599,#9600,#9601,#9602,#9603,#9604,#9605,
#9606,#9607,#9608,#9609,#9610,#9611,#9612,#9613,#9614,#9615,#9616,#9617,
#9618,#9619,#9620,#9621,#9622,#9623,#9624,#9625));
#10376=AXIS2_PLACEMENT_3D('',#23574,#11673,#11674);
#10377=AXIS2_PLACEMENT_3D('',#23575,#11675,#11676);
#10378=AXIS2_PLACEMENT_3D('',#23578,#11677,#11678);
#10379=AXIS2_PLACEMENT_3D('',#23582,#11680,#11681);
#10380=AXIS2_PLACEMENT_3D('',#23584,#11683,#11684);
#10381=AXIS2_PLACEMENT_3D('',#23590,#11688,#11689);
#10382=AXIS2_PLACEMENT_3D('',#23593,#11690,#11691);
#10383=AXIS2_PLACEMENT_3D('',#23597,#11693,#11694);
#10384=AXIS2_PLACEMENT_3D('',#23599,#11696,#11697);
#10385=AXIS2_PLACEMENT_3D('',#23602,#11700,#11701);
#10386=AXIS2_PLACEMENT_3D('',#23604,#11702,#11703);
#10387=AXIS2_PLACEMENT_3D('',#23607,#11705,#11706);
#10388=AXIS2_PLACEMENT_3D('',#23608,#11707,#11708);
#10389=AXIS2_PLACEMENT_3D('',#23614,#11712,#11713);
#10390=AXIS2_PLACEMENT_3D('',#23616,#11714,#11715);
#10391=AXIS2_PLACEMENT_3D('',#23619,#11717,#11718);
#10392=AXIS2_PLACEMENT_3D('',#23620,#11719,#11720);
#10393=AXIS2_PLACEMENT_3D('',#23623,#11723,#11724);
#10394=AXIS2_PLACEMENT_3D('',#23626,#11725,#11726);
#10395=AXIS2_PLACEMENT_3D('',#23630,#11728,#11729);
#10396=AXIS2_PLACEMENT_3D('',#23632,#11731,#11732);
#10397=AXIS2_PLACEMENT_3D('',#23638,#11736,#11737);
#10398=AXIS2_PLACEMENT_3D('',#23641,#11738,#11739);
#10399=AXIS2_PLACEMENT_3D('',#23645,#11741,#11742);
#10400=AXIS2_PLACEMENT_3D('',#23647,#11744,#11745);
#10401=AXIS2_PLACEMENT_3D('',#23650,#11748,#11749);
#10402=AXIS2_PLACEMENT_3D('',#23652,#11750,#11751);
#10403=AXIS2_PLACEMENT_3D('',#23655,#11753,#11754);
#10404=AXIS2_PLACEMENT_3D('',#23656,#11755,#11756);
#10405=AXIS2_PLACEMENT_3D('',#23662,#11760,#11761);
#10406=AXIS2_PLACEMENT_3D('',#23664,#11762,#11763);
#10407=AXIS2_PLACEMENT_3D('',#23667,#11765,#11766);
#10408=AXIS2_PLACEMENT_3D('',#23668,#11767,#11768);
#10409=AXIS2_PLACEMENT_3D('',#23671,#11771,#11772);
#10410=AXIS2_PLACEMENT_3D('',#23674,#11773,#11774);
#10411=AXIS2_PLACEMENT_3D('',#23678,#11776,#11777);
#10412=AXIS2_PLACEMENT_3D('',#23680,#11779,#11780);
#10413=AXIS2_PLACEMENT_3D('',#23686,#11784,#11785);
#10414=AXIS2_PLACEMENT_3D('',#23689,#11786,#11787);
#10415=AXIS2_PLACEMENT_3D('',#23693,#11789,#11790);
#10416=AXIS2_PLACEMENT_3D('',#23695,#11792,#11793);
#10417=AXIS2_PLACEMENT_3D('',#23698,#11796,#11797);
#10418=AXIS2_PLACEMENT_3D('',#23700,#11798,#11799);
#10419=AXIS2_PLACEMENT_3D('',#23703,#11801,#11802);
#10420=AXIS2_PLACEMENT_3D('',#23704,#11803,#11804);
#10421=AXIS2_PLACEMENT_3D('',#23710,#11808,#11809);
#10422=AXIS2_PLACEMENT_3D('',#23712,#11810,#11811);
#10423=AXIS2_PLACEMENT_3D('',#23715,#11813,#11814);
#10424=AXIS2_PLACEMENT_3D('',#23716,#11815,#11816);
#10425=AXIS2_PLACEMENT_3D('',#23719,#11819,#11820);
#10426=AXIS2_PLACEMENT_3D('',#23721,#11821,#11822);
#10427=AXIS2_PLACEMENT_3D('',#23724,#11824,#11825);
#10428=AXIS2_PLACEMENT_3D('',#23725,#11826,#11827);
#10429=AXIS2_PLACEMENT_3D('',#23727,#11828,#11829);
#10430=AXIS2_PLACEMENT_3D('',#23730,#11831,#11832);
#10431=AXIS2_PLACEMENT_3D('',#23731,#11833,#11834);
#10432=AXIS2_PLACEMENT_3D('',#23733,#11835,#11836);
#10433=AXIS2_PLACEMENT_3D('',#23736,#11838,#11839);
#10434=AXIS2_PLACEMENT_3D('',#23737,#11840,#11841);
#10435=AXIS2_PLACEMENT_3D('',#23739,#11842,#11843);
#10436=AXIS2_PLACEMENT_3D('',#23742,#11845,#11846);
#10437=AXIS2_PLACEMENT_3D('',#23743,#11847,#11848);
#10438=AXIS2_PLACEMENT_3D('',#23745,#11849,#11850);
#10439=AXIS2_PLACEMENT_3D('',#23748,#11852,#11853);
#10440=AXIS2_PLACEMENT_3D('',#23749,#11854,#11855);
#10441=AXIS2_PLACEMENT_3D('',#23751,#11856,#11857);
#10442=AXIS2_PLACEMENT_3D('',#23754,#11859,#11860);
#10443=AXIS2_PLACEMENT_3D('',#23755,#11861,#11862);
#10444=AXIS2_PLACEMENT_3D('',#23764,#11867,#11868);
#10445=AXIS2_PLACEMENT_3D('',#23770,#11872,#11873);
#10446=AXIS2_PLACEMENT_3D('',#23776,#11877,#11878);
#10447=AXIS2_PLACEMENT_3D('',#23782,#11882,#11883);
#10448=AXIS2_PLACEMENT_3D('',#23788,#11887,#11888);
#10449=AXIS2_PLACEMENT_3D('',#23794,#11892,#11893);
#10450=AXIS2_PLACEMENT_3D('',#23800,#11897,#11898);
#10451=AXIS2_PLACEMENT_3D('',#23803,#11901,#11902);
#10452=AXIS2_PLACEMENT_3D('',#23804,#11903,#11904);
#11673=DIRECTION('axis',(0.,0.,1.));
#11674=DIRECTION('refdir',(1.,0.,0.));
#11675=DIRECTION('center_axis',(0.,1.,0.));
#11676=DIRECTION('ref_axis',(0.707106781186548,0.,0.707106781186548));
#11677=DIRECTION('center_axis',(0.,-1.,0.));
#11678=DIRECTION('ref_axis',(0.707106781186548,0.,0.707106781186548));
#11679=DIRECTION('',(0.,1.,0.));
#11680=DIRECTION('center_axis',(0.,1.,0.));
#11681=DIRECTION('ref_axis',(0.707106781186548,0.,0.707106781186548));
#11682=DIRECTION('',(0.,-1.,0.));
#11683=DIRECTION('center_axis',(0.,0.,1.));
#11684=DIRECTION('ref_axis',(1.,0.,0.));
#11685=DIRECTION('',(1.,0.,0.));
#11686=DIRECTION('',(0.,-1.,0.));
#11687=DIRECTION('',(-1.,0.,0.));
#11688=DIRECTION('center_axis',(0.,1.,0.));
#11689=DIRECTION('ref_axis',(0.707106781186549,0.,-0.707106781186546));
#11690=DIRECTION('center_axis',(0.,-1.,0.));
#11691=DIRECTION('ref_axis',(0.707106781186549,0.,-0.707106781186546));
#11692=DIRECTION('',(0.,1.,0.));
#11693=DIRECTION('center_axis',(0.,1.,0.));
#11694=DIRECTION('ref_axis',(0.707106781186549,0.,-0.707106781186546));
#11695=DIRECTION('',(0.,-1.,0.));
#11696=DIRECTION('center_axis',(1.,0.,0.));
#11697=DIRECTION('ref_axis',(0.,0.,-1.));
#11698=DIRECTION('',(0.,0.,1.));
#11699=DIRECTION('',(0.,0.,-1.));
#11700=DIRECTION('center_axis',(0.,1.,0.));
#11701=DIRECTION('ref_axis',(-0.707106781186548,0.,0.707106781186547));
#11702=DIRECTION('center_axis',(0.,-1.,0.));
#11703=DIRECTION('ref_axis',(-0.707106781186548,0.,0.707106781186547));
#11704=DIRECTION('',(0.,1.,0.));
#11705=DIRECTION('center_axis',(0.,1.,0.));
#11706=DIRECTION('ref_axis',(-0.707106781186548,0.,0.707106781186547));
#11707=DIRECTION('center_axis',(-1.,0.,0.));
#11708=DIRECTION('ref_axis',(0.,0.,1.));
#11709=DIRECTION('',(0.,0.,1.));
#11710=DIRECTION('',(0.,-1.,0.));
#11711=DIRECTION('',(0.,0.,-1.));
#11712=DIRECTION('center_axis',(0.,1.,0.));
#11713=DIRECTION('ref_axis',(-0.707106781186545,0.,-0.70710678118655));
#11714=DIRECTION('center_axis',(0.,-1.,0.));
#11715=DIRECTION('ref_axis',(-0.707106781186545,0.,-0.70710678118655));
#11716=DIRECTION('',(0.,1.,0.));
#11717=DIRECTION('center_axis',(0.,1.,0.));
#11718=DIRECTION('ref_axis',(-0.707106781186545,0.,-0.70710678118655));
#11719=DIRECTION('center_axis',(0.,0.,-1.));
#11720=DIRECTION('ref_axis',(-1.,0.,0.));
#11721=DIRECTION('',(1.,0.,0.));
#11722=DIRECTION('',(-1.,0.,0.));
#11723=DIRECTION('center_axis',(0.,1.,0.));
#11724=DIRECTION('ref_axis',(0.707106781186548,0.,-0.707106781186547));
#11725=DIRECTION('center_axis',(0.,-1.,0.));
#11726=DIRECTION('ref_axis',(0.707106781186548,0.,-0.707106781186547));
#11727=DIRECTION('',(0.,1.,0.));
#11728=DIRECTION('center_axis',(0.,1.,0.));
#11729=DIRECTION('ref_axis',(0.707106781186548,0.,-0.707106781186547));
#11730=DIRECTION('',(0.,-1.,0.));
#11731=DIRECTION('center_axis',(1.,0.,0.));
#11732=DIRECTION('ref_axis',(0.,0.,-1.));
#11733=DIRECTION('',(0.,0.,-1.));
#11734=DIRECTION('',(0.,-1.,0.));
#11735=DIRECTION('',(0.,0.,1.));
#11736=DIRECTION('center_axis',(0.,1.,0.));
#11737=DIRECTION('ref_axis',(-0.707106781186544,0.,-0.707106781186551));
#11738=DIRECTION('center_axis',(0.,-1.,0.));
#11739=DIRECTION('ref_axis',(-0.707106781186544,0.,-0.707106781186551));
#11740=DIRECTION('',(0.,1.,0.));
#11741=DIRECTION('center_axis',(0.,1.,0.));
#11742=DIRECTION('ref_axis',(-0.707106781186544,0.,-0.707106781186551));
#11743=DIRECTION('',(0.,-1.,0.));
#11744=DIRECTION('center_axis',(0.,0.,-1.));
#11745=DIRECTION('ref_axis',(-1.,0.,0.));
#11746=DIRECTION('',(1.,0.,0.));
#11747=DIRECTION('',(-1.,0.,0.));
#11748=DIRECTION('center_axis',(0.,1.,0.));
#11749=DIRECTION('ref_axis',(0.707106781186548,0.,0.707106781186547));
#11750=DIRECTION('center_axis',(0.,-1.,0.));
#11751=DIRECTION('ref_axis',(0.707106781186548,0.,0.707106781186547));
#11752=DIRECTION('',(0.,1.,0.));
#11753=DIRECTION('center_axis',(0.,1.,0.));
#11754=DIRECTION('ref_axis',(0.707106781186548,0.,0.707106781186547));
#11755=DIRECTION('center_axis',(0.,0.,1.));
#11756=DIRECTION('ref_axis',(1.,0.,0.));
#11757=DIRECTION('',(1.,0.,0.));
#11758=DIRECTION('',(0.,-1.,0.));
#11759=DIRECTION('',(-1.,0.,0.));
#11760=DIRECTION('center_axis',(0.,1.,0.));
#11761=DIRECTION('ref_axis',(-0.707106781186549,0.,0.707106781186546));
#11762=DIRECTION('center_axis',(0.,-1.,0.));
#11763=DIRECTION('ref_axis',(-0.707106781186549,0.,0.707106781186546));
#11764=DIRECTION('',(0.,1.,0.));
#11765=DIRECTION('center_axis',(0.,1.,0.));
#11766=DIRECTION('ref_axis',(-0.707106781186549,0.,0.707106781186546));
#11767=DIRECTION('center_axis',(-1.,0.,0.));
#11768=DIRECTION('ref_axis',(0.,0.,1.));
#11769=DIRECTION('',(0.,0.,-1.));
#11770=DIRECTION('',(0.,0.,1.));
#11771=DIRECTION('center_axis',(0.,1.,0.));
#11772=DIRECTION('ref_axis',(0.707106781186549,0.,0.707106781186546));
#11773=DIRECTION('center_axis',(0.,-1.,0.));
#11774=DIRECTION('ref_axis',(0.707106781186549,0.,0.707106781186546));
#11775=DIRECTION('',(0.,1.,0.));
#11776=DIRECTION('center_axis',(0.,1.,0.));
#11777=DIRECTION('ref_axis',(0.707106781186549,0.,0.707106781186546));
#11778=DIRECTION('',(0.,-1.,0.));
#11779=DIRECTION('center_axis',(0.,0.,1.));
#11780=DIRECTION('ref_axis',(1.,0.,0.));
#11781=DIRECTION('',(1.,0.,0.));
#11782=DIRECTION('',(0.,-1.,0.));
#11783=DIRECTION('',(-1.,0.,0.));
#11784=DIRECTION('center_axis',(0.,1.,0.));
#11785=DIRECTION('ref_axis',(0.707106781186549,0.,-0.707106781186546));
#11786=DIRECTION('center_axis',(0.,-1.,0.));
#11787=DIRECTION('ref_axis',(0.707106781186549,0.,-0.707106781186546));
#11788=DIRECTION('',(0.,1.,0.));
#11789=DIRECTION('center_axis',(0.,1.,0.));
#11790=DIRECTION('ref_axis',(0.707106781186549,0.,-0.707106781186546));
#11791=DIRECTION('',(0.,-1.,0.));
#11792=DIRECTION('center_axis',(1.,0.,0.));
#11793=DIRECTION('ref_axis',(0.,0.,-1.));
#11794=DIRECTION('',(0.,0.,1.));
#11795=DIRECTION('',(0.,0.,-1.));
#11796=DIRECTION('center_axis',(0.,1.,0.));
#11797=DIRECTION('ref_axis',(-0.707106781186549,0.,0.707106781186546));
#11798=DIRECTION('center_axis',(0.,-1.,0.));
#11799=DIRECTION('ref_axis',(-0.707106781186549,0.,0.707106781186546));
#11800=DIRECTION('',(0.,1.,0.));
#11801=DIRECTION('center_axis',(0.,1.,0.));
#11802=DIRECTION('ref_axis',(-0.707106781186549,0.,0.707106781186546));
#11803=DIRECTION('center_axis',(-1.,0.,0.));
#11804=DIRECTION('ref_axis',(0.,0.,1.));
#11805=DIRECTION('',(0.,0.,1.));
#11806=DIRECTION('',(0.,-1.,0.));
#11807=DIRECTION('',(0.,0.,-1.));
#11808=DIRECTION('center_axis',(0.,1.,0.));
#11809=DIRECTION('ref_axis',(-0.707106781186546,0.,-0.707106781186549));
#11810=DIRECTION('center_axis',(0.,-1.,0.));
#11811=DIRECTION('ref_axis',(-0.707106781186546,0.,-0.707106781186549));
#11812=DIRECTION('',(0.,1.,0.));
#11813=DIRECTION('center_axis',(0.,1.,0.));
#11814=DIRECTION('ref_axis',(-0.707106781186546,0.,-0.707106781186549));
#11815=DIRECTION('center_axis',(0.,0.,-1.));
#11816=DIRECTION('ref_axis',(-1.,0.,0.));
#11817=DIRECTION('',(1.,0.,0.));
#11818=DIRECTION('',(-1.,0.,0.));
#11819=DIRECTION('center_axis',(0.,1.,0.));
#11820=DIRECTION('ref_axis',(1.,0.,0.));
#11821=DIRECTION('center_axis',(0.,1.,0.));
#11822=DIRECTION('ref_axis',(1.,0.,0.));
#11823=DIRECTION('',(0.,1.,0.));
#11824=DIRECTION('center_axis',(0.,-1.,0.));
#11825=DIRECTION('ref_axis',(1.,0.,0.));
#11826=DIRECTION('center_axis',(0.,1.,0.));
#11827=DIRECTION('ref_axis',(1.,0.,0.));
#11828=DIRECTION('center_axis',(0.,1.,0.));
#11829=DIRECTION('ref_axis',(1.,0.,0.));
#11830=DIRECTION('',(0.,1.,0.));
#11831=DIRECTION('center_axis',(0.,-1.,0.));
#11832=DIRECTION('ref_axis',(1.,0.,0.));
#11833=DIRECTION('center_axis',(0.,1.,0.));
#11834=DIRECTION('ref_axis',(1.,0.,0.));
#11835=DIRECTION('center_axis',(0.,1.,0.));
#11836=DIRECTION('ref_axis',(1.,0.,0.));
#11837=DIRECTION('',(0.,1.,0.));
#11838=DIRECTION('center_axis',(0.,-1.,0.));
#11839=DIRECTION('ref_axis',(1.,0.,0.));
#11840=DIRECTION('center_axis',(0.,1.,0.));
#11841=DIRECTION('ref_axis',(1.,0.,0.));
#11842=DIRECTION('center_axis',(0.,1.,0.));
#11843=DIRECTION('ref_axis',(1.,0.,0.));
#11844=DIRECTION('',(0.,1.,0.));
#11845=DIRECTION('center_axis',(0.,-1.,0.));
#11846=DIRECTION('ref_axis',(1.,0.,0.));
#11847=DIRECTION('center_axis',(0.,1.,0.));
#11848=DIRECTION('ref_axis',(1.,0.,0.));
#11849=DIRECTION('center_axis',(0.,1.,0.));
#11850=DIRECTION('ref_axis',(1.,0.,0.));
#11851=DIRECTION('',(0.,1.,0.));
#11852=DIRECTION('center_axis',(0.,-1.,0.));
#11853=DIRECTION('ref_axis',(1.,0.,0.));
#11854=DIRECTION('center_axis',(0.,1.,0.));
#11855=DIRECTION('ref_axis',(1.,0.,0.));
#11856=DIRECTION('center_axis',(0.,1.,0.));
#11857=DIRECTION('ref_axis',(1.,0.,0.));
#11858=DIRECTION('',(0.,1.,0.));
#11859=DIRECTION('center_axis',(0.,-1.,0.));
#11860=DIRECTION('ref_axis',(1.,0.,0.));
#11861=DIRECTION('center_axis',(-1.,0.,0.));
#11862=DIRECTION('ref_axis',(0.,0.,1.));
#11863=DIRECTION('',(0.,0.,-1.));
#11864=DIRECTION('',(0.,1.,0.));
#11865=DIRECTION('',(0.,0.,1.));
#11866=DIRECTION('',(0.,1.,0.));
#11867=DIRECTION('center_axis',(0.,0.,-1.));
#11868=DIRECTION('ref_axis',(-1.,0.,0.));
#11869=DIRECTION('',(1.,0.,0.));
#11870=DIRECTION('',(-1.,0.,0.));
#11871=DIRECTION('',(0.,1.,0.));
#11872=DIRECTION('center_axis',(1.,0.,0.));
#11873=DIRECTION('ref_axis',(0.,0.,-1.));
#11874=DIRECTION('',(0.,0.,1.));
#11875=DIRECTION('',(0.,0.,-1.));
#11876=DIRECTION('',(0.,1.,0.));
#11877=DIRECTION('center_axis',(0.936329177569044,0.,0.351123441588392));
#11878=DIRECTION('ref_axis',(0.351123441588392,0.,-0.936329177569044));
#11879=DIRECTION('',(-0.351123441588392,0.,0.936329177569044));
#11880=DIRECTION('',(0.351123441588392,0.,-0.936329177569044));
#11881=DIRECTION('',(0.,1.,0.));
#11882=DIRECTION('center_axis',(0.6,0.,0.8));
#11883=DIRECTION('ref_axis',(0.8,0.,-0.6));
#11884=DIRECTION('',(-0.8,0.,0.6));
#11885=DIRECTION('',(0.8,0.,-0.6));
#11886=DIRECTION('',(0.,1.,0.));
#11887=DIRECTION('center_axis',(0.,0.,1.));
#11888=DIRECTION('ref_axis',(1.,0.,0.));
#11889=DIRECTION('',(-1.,0.,0.));
#11890=DIRECTION('',(1.,0.,0.));
#11891=DIRECTION('',(0.,1.,0.));
#11892=DIRECTION('center_axis',(-0.6,0.,0.8));
#11893=DIRECTION('ref_axis',(0.8,0.,0.6));
#11894=DIRECTION('',(-0.8,0.,-0.6));
#11895=DIRECTION('',(0.8,0.,0.6));
#11896=DIRECTION('',(0.,1.,0.));
#11897=DIRECTION('center_axis',(-0.936329177569044,0.,0.351123441588392));
#11898=DIRECTION('ref_axis',(0.351123441588392,0.,0.936329177569044));
#11899=DIRECTION('',(-0.351123441588392,0.,-0.936329177569044));
#11900=DIRECTION('',(0.351123441588392,0.,0.936329177569044));
#11901=DIRECTION('center_axis',(0.,1.,0.));
#11902=DIRECTION('ref_axis',(0.,0.,1.));
#11903=DIRECTION('center_axis',(0.,1.,0.));
#11904=DIRECTION('ref_axis',(1.,0.,0.));
#23574=CARTESIAN_POINT('',(0.,0.,0.));
#23575=CARTESIAN_POINT('Origin',(2.9,3.7,9.1));
#23576=CARTESIAN_POINT('',(3.1,3.7,9.1));
#23577=CARTESIAN_POINT('',(2.9,3.7,9.3));
#23578=CARTESIAN_POINT('Origin',(2.9,3.7,9.1));
#23579=CARTESIAN_POINT('',(2.9,3.85,9.3));
#23580=CARTESIAN_POINT('',(2.9,3.7,9.3));
#23581=CARTESIAN_POINT('',(3.1,3.85,9.1));
#23582=CARTESIAN_POINT('Origin',(2.9,3.85,9.1));
#23583=CARTESIAN_POINT('',(3.1,3.7,9.1));
#23584=CARTESIAN_POINT('Origin',(1.5,3.7,9.3));
#23585=CARTESIAN_POINT('',(1.7,3.7,9.3));
#23586=CARTESIAN_POINT('',(0.75,3.7,9.3));
#23587=CARTESIAN_POINT('',(1.7,3.85,9.3));
#23588=CARTESIAN_POINT('',(1.7,3.7,9.3));
#23589=CARTESIAN_POINT('',(0.75,3.85,9.3));
#23590=CARTESIAN_POINT('Origin',(2.9,3.7,4.2));
#23591=CARTESIAN_POINT('',(2.9,3.7,4.));
#23592=CARTESIAN_POINT('',(3.1,3.7,4.2));
#23593=CARTESIAN_POINT('Origin',(2.9,3.7,4.2));
#23594=CARTESIAN_POINT('',(3.1,3.85,4.2));
#23595=CARTESIAN_POINT('',(3.1,3.7,4.2));
#23596=CARTESIAN_POINT('',(2.9,3.85,4.));
#23597=CARTESIAN_POINT('Origin',(2.9,3.85,4.2));
#23598=CARTESIAN_POINT('',(2.9,3.7,4.));
#23599=CARTESIAN_POINT('Origin',(3.1,3.7,9.3));
#23600=CARTESIAN_POINT('',(3.1,3.85,8.25));
#23601=CARTESIAN_POINT('',(3.1,3.7,8.25));
#23602=CARTESIAN_POINT('Origin',(1.7,3.7,9.1));
#23603=CARTESIAN_POINT('',(1.5,3.7,9.1));
#23604=CARTESIAN_POINT('Origin',(1.7,3.7,9.1));
#23605=CARTESIAN_POINT('',(1.5,3.85,9.1));
#23606=CARTESIAN_POINT('',(1.5,3.7,9.1));
#23607=CARTESIAN_POINT('Origin',(1.7,3.85,9.1));
#23608=CARTESIAN_POINT('Origin',(1.5,3.7,4.));
#23609=CARTESIAN_POINT('',(1.5,3.7,4.2));
#23610=CARTESIAN_POINT('',(1.5,3.7,5.6));
#23611=CARTESIAN_POINT('',(1.5,3.85,4.2));
#23612=CARTESIAN_POINT('',(1.5,3.7,4.2));
#23613=CARTESIAN_POINT('',(1.5,3.85,5.6));
#23614=CARTESIAN_POINT('Origin',(1.7,3.7,4.2));
#23615=CARTESIAN_POINT('',(1.7,3.7,4.));
#23616=CARTESIAN_POINT('Origin',(1.7,3.7,4.2));
#23617=CARTESIAN_POINT('',(1.7,3.85,4.));
#23618=CARTESIAN_POINT('',(1.7,3.7,4.));
#23619=CARTESIAN_POINT('Origin',(1.7,3.85,4.2));
#23620=CARTESIAN_POINT('Origin',(3.1,3.7,4.));
#23621=CARTESIAN_POINT('',(1.55,3.85,4.));
#23622=CARTESIAN_POINT('',(1.55,3.7,4.));
#23623=CARTESIAN_POINT('Origin',(-1.7,3.7,4.2));
#23624=CARTESIAN_POINT('',(-1.7,3.7,4.));
#23625=CARTESIAN_POINT('',(-1.5,3.7,4.2));
#23626=CARTESIAN_POINT('Origin',(-1.7,3.7,4.2));
#23627=CARTESIAN_POINT('',(-1.5,3.85,4.2));
#23628=CARTESIAN_POINT('',(-1.5,3.7,4.2));
#23629=CARTESIAN_POINT('',(-1.7,3.85,4.));
#23630=CARTESIAN_POINT('Origin',(-1.7,3.85,4.2));
#23631=CARTESIAN_POINT('',(-1.7,3.7,4.));
#23632=CARTESIAN_POINT('Origin',(-1.5,3.7,9.3));
#23633=CARTESIAN_POINT('',(-1.5,3.7,9.1));
#23634=CARTESIAN_POINT('',(-1.5,3.7,8.25));
#23635=CARTESIAN_POINT('',(-1.5,3.85,9.1));
#23636=CARTESIAN_POINT('',(-1.5,3.7,9.1));
#23637=CARTESIAN_POINT('',(-1.5,3.85,8.25));
#23638=CARTESIAN_POINT('Origin',(-2.9,3.7,4.2));
#23639=CARTESIAN_POINT('',(-3.1,3.7,4.2));
#23640=CARTESIAN_POINT('',(-2.9,3.7,4.));
#23641=CARTESIAN_POINT('Origin',(-2.9,3.7,4.2));
#23642=CARTESIAN_POINT('',(-2.9,3.85,4.));
#23643=CARTESIAN_POINT('',(-2.9,3.7,4.));
#23644=CARTESIAN_POINT('',(-3.1,3.85,4.2));
#23645=CARTESIAN_POINT('Origin',(-2.9,3.85,4.2));
#23646=CARTESIAN_POINT('',(-3.1,3.7,4.2));
#23647=CARTESIAN_POINT('Origin',(-1.5,3.7,4.));
#23648=CARTESIAN_POINT('',(-0.75,3.85,4.));
#23649=CARTESIAN_POINT('',(-0.75,3.7,4.));
#23650=CARTESIAN_POINT('Origin',(-1.7,3.7,9.1));
#23651=CARTESIAN_POINT('',(-1.7,3.7,9.3));
#23652=CARTESIAN_POINT('Origin',(-1.7,3.7,9.1));
#23653=CARTESIAN_POINT('',(-1.7,3.85,9.3));
#23654=CARTESIAN_POINT('',(-1.7,3.7,9.3));
#23655=CARTESIAN_POINT('Origin',(-1.7,3.85,9.1));
#23656=CARTESIAN_POINT('Origin',(-3.1,3.7,9.3));
#23657=CARTESIAN_POINT('',(-2.9,3.7,9.3));
#23658=CARTESIAN_POINT('',(-1.55,3.7,9.3));
#23659=CARTESIAN_POINT('',(-2.9,3.85,9.3));
#23660=CARTESIAN_POINT('',(-2.9,3.7,9.3));
#23661=CARTESIAN_POINT('',(-1.55,3.85,9.3));
#23662=CARTESIAN_POINT('Origin',(-2.9,3.7,9.1));
#23663=CARTESIAN_POINT('',(-3.1,3.7,9.1));
#23664=CARTESIAN_POINT('Origin',(-2.9,3.7,9.1));
#23665=CARTESIAN_POINT('',(-3.1,3.85,9.1));
#23666=CARTESIAN_POINT('',(-3.1,3.7,9.1));
#23667=CARTESIAN_POINT('Origin',(-2.9,3.85,9.1));
#23668=CARTESIAN_POINT('Origin',(-3.1,3.7,4.));
#23669=CARTESIAN_POINT('',(-3.1,3.85,5.6));
#23670=CARTESIAN_POINT('',(-3.1,3.7,5.6));
#23671=CARTESIAN_POINT('Origin',(1.1,3.7,12.));
#23672=CARTESIAN_POINT('',(1.3,3.7,12.));
#23673=CARTESIAN_POINT('',(1.1,3.7,12.2));
#23674=CARTESIAN_POINT('Origin',(1.1,3.7,12.));
#23675=CARTESIAN_POINT('',(1.1,3.85,12.2));
#23676=CARTESIAN_POINT('',(1.1,3.7,12.2));
#23677=CARTESIAN_POINT('',(1.3,3.85,12.));
#23678=CARTESIAN_POINT('Origin',(1.1,3.85,12.));
#23679=CARTESIAN_POINT('',(1.3,3.7,12.));
#23680=CARTESIAN_POINT('Origin',(-1.3,3.7,12.2));
#23681=CARTESIAN_POINT('',(-1.1,3.7,12.2));
#23682=CARTESIAN_POINT('',(-0.65,3.7,12.2));
#23683=CARTESIAN_POINT('',(-1.1,3.85,12.2));
#23684=CARTESIAN_POINT('',(-1.1,3.7,12.2));
#23685=CARTESIAN_POINT('',(-0.65,3.85,12.2));
#23686=CARTESIAN_POINT('Origin',(1.1,3.7,4.2));
#23687=CARTESIAN_POINT('',(1.1,3.7,4.));
#23688=CARTESIAN_POINT('',(1.3,3.7,4.2));
#23689=CARTESIAN_POINT('Origin',(1.1,3.7,4.2));
#23690=CARTESIAN_POINT('',(1.3,3.85,4.2));
#23691=CARTESIAN_POINT('',(1.3,3.7,4.2));
#23692=CARTESIAN_POINT('',(1.1,3.85,4.));
#23693=CARTESIAN_POINT('Origin',(1.1,3.85,4.2));
#23694=CARTESIAN_POINT('',(1.1,3.7,4.));
#23695=CARTESIAN_POINT('Origin',(1.3,3.7,12.2));
#23696=CARTESIAN_POINT('',(1.3,3.85,9.7));
#23697=CARTESIAN_POINT('',(1.3,3.7,9.7));
#23698=CARTESIAN_POINT('Origin',(-1.1,3.7,12.));
#23699=CARTESIAN_POINT('',(-1.3,3.7,12.));
#23700=CARTESIAN_POINT('Origin',(-1.1,3.7,12.));
#23701=CARTESIAN_POINT('',(-1.3,3.85,12.));
#23702=CARTESIAN_POINT('',(-1.3,3.7,12.));
#23703=CARTESIAN_POINT('Origin',(-1.1,3.85,12.));
#23704=CARTESIAN_POINT('Origin',(-1.3,3.7,4.));
#23705=CARTESIAN_POINT('',(-1.3,3.7,4.2));
#23706=CARTESIAN_POINT('',(-1.3,3.7,5.6));
#23707=CARTESIAN_POINT('',(-1.3,3.85,4.2));
#23708=CARTESIAN_POINT('',(-1.3,3.7,4.2));
#23709=CARTESIAN_POINT('',(-1.3,3.85,5.6));
#23710=CARTESIAN_POINT('Origin',(-1.1,3.7,4.2));
#23711=CARTESIAN_POINT('',(-1.1,3.7,4.));
#23712=CARTESIAN_POINT('Origin',(-1.1,3.7,4.2));
#23713=CARTESIAN_POINT('',(-1.1,3.85,4.));
#23714=CARTESIAN_POINT('',(-1.1,3.7,4.));
#23715=CARTESIAN_POINT('Origin',(-1.1,3.85,4.2));
#23716=CARTESIAN_POINT('Origin',(1.3,3.7,4.));
#23717=CARTESIAN_POINT('',(0.65,3.85,4.));
#23718=CARTESIAN_POINT('',(0.65,3.7,4.));
#23719=CARTESIAN_POINT('Origin',(3.55,3.7,10.));
#23720=CARTESIAN_POINT('',(3.325,3.7,10.));
#23721=CARTESIAN_POINT('Origin',(3.55,3.7,10.));
#23722=CARTESIAN_POINT('',(3.325,3.85,10.));
#23723=CARTESIAN_POINT('',(3.325,3.7,10.));
#23724=CARTESIAN_POINT('Origin',(3.55,3.85,10.));
#23725=CARTESIAN_POINT('Origin',(3.,3.7,11.7));
#23726=CARTESIAN_POINT('',(2.64,3.7,11.7));
#23727=CARTESIAN_POINT('Origin',(3.,3.7,11.7));
#23728=CARTESIAN_POINT('',(2.64,3.85,11.7));
#23729=CARTESIAN_POINT('',(2.64,3.7,11.7));
#23730=CARTESIAN_POINT('Origin',(3.,3.85,11.7));
#23731=CARTESIAN_POINT('Origin',(-3.,3.7,11.7));
#23732=CARTESIAN_POINT('',(-3.36,3.7,11.7));
#23733=CARTESIAN_POINT('Origin',(-3.,3.7,11.7));
#23734=CARTESIAN_POINT('',(-3.36,3.85,11.7));
#23735=CARTESIAN_POINT('',(-3.36,3.7,11.7));
#23736=CARTESIAN_POINT('Origin',(-3.,3.85,11.7));
#23737=CARTESIAN_POINT('Origin',(3.55,3.7,2.5));
#23738=CARTESIAN_POINT('',(3.325,3.7,2.5));
#23739=CARTESIAN_POINT('Origin',(3.55,3.7,2.5));
#23740=CARTESIAN_POINT('',(3.325,3.85,2.5));
#23741=CARTESIAN_POINT('',(3.325,3.7,2.5));
#23742=CARTESIAN_POINT('Origin',(3.55,3.85,2.5));
#23743=CARTESIAN_POINT('Origin',(-3.55,3.7,2.5));
#23744=CARTESIAN_POINT('',(-3.775,3.7,2.5));
#23745=CARTESIAN_POINT('Origin',(-3.55,3.7,2.5));
#23746=CARTESIAN_POINT('',(-3.775,3.85,2.5));
#23747=CARTESIAN_POINT('',(-3.775,3.7,2.5));
#23748=CARTESIAN_POINT('Origin',(-3.55,3.85,2.5));
#23749=CARTESIAN_POINT('Origin',(-3.55,3.7,10.));
#23750=CARTESIAN_POINT('',(-3.775,3.7,10.));
#23751=CARTESIAN_POINT('Origin',(-3.55,3.7,10.));
#23752=CARTESIAN_POINT('',(-3.775,3.85,10.));
#23753=CARTESIAN_POINT('',(-3.775,3.7,10.));
#23754=CARTESIAN_POINT('Origin',(-3.55,3.85,10.));
#23755=CARTESIAN_POINT('Origin',(-3.9,3.7,1.7));
#23756=CARTESIAN_POINT('',(-3.9,3.7,11.3));
#23757=CARTESIAN_POINT('',(-3.9,3.7,1.7));
#23758=CARTESIAN_POINT('',(-3.9,3.7,11.3));
#23759=CARTESIAN_POINT('',(-3.9,3.85,11.3));
#23760=CARTESIAN_POINT('',(-3.9,3.7,11.3));
#23761=CARTESIAN_POINT('',(-3.9,3.85,1.7));
#23762=CARTESIAN_POINT('',(-3.9,3.85,11.3));
#23763=CARTESIAN_POINT('',(-3.9,3.7,1.7));
#23764=CARTESIAN_POINT('Origin',(3.9,3.7,1.7));
#23765=CARTESIAN_POINT('',(3.9,3.7,1.7));
#23766=CARTESIAN_POINT('',(-3.9,3.7,1.7));
#23767=CARTESIAN_POINT('',(3.9,3.85,1.7));
#23768=CARTESIAN_POINT('',(-3.9,3.85,1.7));
#23769=CARTESIAN_POINT('',(3.9,3.7,1.7));
#23770=CARTESIAN_POINT('Origin',(3.9,3.7,11.3));
#23771=CARTESIAN_POINT('',(3.9,3.7,11.3));
#23772=CARTESIAN_POINT('',(3.9,3.7,1.7));
#23773=CARTESIAN_POINT('',(3.9,3.85,11.3));
#23774=CARTESIAN_POINT('',(3.9,3.85,1.7));
#23775=CARTESIAN_POINT('',(3.9,3.7,11.3));
#23776=CARTESIAN_POINT('Origin',(3.6,3.7,12.1));
#23777=CARTESIAN_POINT('',(3.6,3.7,12.1));
#23778=CARTESIAN_POINT('',(3.9,3.7,11.3));
#23779=CARTESIAN_POINT('',(3.6,3.85,12.1));
#23780=CARTESIAN_POINT('',(3.9,3.85,11.3));
#23781=CARTESIAN_POINT('',(3.6,3.7,12.1));
#23782=CARTESIAN_POINT('Origin',(2.8,3.7,12.7));
#23783=CARTESIAN_POINT('',(2.8,3.7,12.7));
#23784=CARTESIAN_POINT('',(3.6,3.7,12.1));
#23785=CARTESIAN_POINT('',(2.8,3.85,12.7));
#23786=CARTESIAN_POINT('',(3.6,3.85,12.1));
#23787=CARTESIAN_POINT('',(2.8,3.7,12.7));
#23788=CARTESIAN_POINT('Origin',(-2.8,3.7,12.7));
#23789=CARTESIAN_POINT('',(-2.8,3.7,12.7));
#23790=CARTESIAN_POINT('',(2.8,3.7,12.7));
#23791=CARTESIAN_POINT('',(-2.8,3.85,12.7));
#23792=CARTESIAN_POINT('',(2.8,3.85,12.7));
#23793=CARTESIAN_POINT('',(-2.8,3.7,12.7));
#23794=CARTESIAN_POINT('Origin',(-3.6,3.7,12.1));
#23795=CARTESIAN_POINT('',(-3.6,3.7,12.1));
#23796=CARTESIAN_POINT('',(-2.8,3.7,12.7));
#23797=CARTESIAN_POINT('',(-3.6,3.85,12.1));
#23798=CARTESIAN_POINT('',(-2.8,3.85,12.7));
#23799=CARTESIAN_POINT('',(-3.6,3.7,12.1));
#23800=CARTESIAN_POINT('Origin',(-3.9,3.7,11.3));
#23801=CARTESIAN_POINT('',(-3.6,3.7,12.1));
#23802=CARTESIAN_POINT('',(-3.6,3.85,12.1));
#23803=CARTESIAN_POINT('Origin',(0.,3.85,7.2));
#23804=CARTESIAN_POINT('Origin',(0.,3.7,7.2));
#85753=UNCERTAINTY_MEASURE_WITH_UNIT(LENGTH_MEASURE(0.001),#85790,
'DISTANCE_ACCURACY_VALUE',
'Maximum model space distance between geometric entities at asserted c
onnectivities');
#85769=UNCERTAINTY_MEASURE_WITH_UNIT(LENGTH_MEASURE(0.001),#85790,
'DISTANCE_ACCURACY_VALUE',
'Maximum model space distance between geometric entities at asserted c
onnectivities');
#85773=(
GEOMETRIC_REPRESENTATION_CONTEXT(3)
GLOBAL_UNCERTAINTY_ASSIGNED_CONTEXT((#85753))
GLOBAL_UNIT_ASSIGNED_CONTEXT((#85790,#85792,#85793))
REPRESENTATION_CONTEXT('','3D')
);
#85789=(
GEOMETRIC_REPRESENTATION_CONTEXT(3)
GLOBAL_UNCERTAINTY_ASSIGNED_CONTEXT((#85769))
GLOBAL_UNIT_ASSIGNED_CONTEXT((#85790,#85792,#85793))
REPRESENTATION_CONTEXT('','3D')
);
#85790=(
LENGTH_UNIT()
NAMED_UNIT(*)
SI_UNIT(.CENTI.,.METRE.)
);
#85792=(
NAMED_UNIT(*)
PLANE_ANGLE_UNIT()
SI_UNIT($,.RADIAN.)
);
#85793=(
NAMED_UNIT(*)
SI_UNIT($,.STERADIAN.)
SOLID_ANGLE_UNIT()
);
#85797=SHAPE_DEFINITION_REPRESENTATION(#85816,#85865);
#85816=PRODUCT_DEFINITION_SHAPE('',$,#85885);
#85865=SHAPE_REPRESENTATION('',(#10376),#85773);
#85881=PRODUCT_DEFINITION_CONTEXT('part definition',#85940,'design');
#85885=PRODUCT_DEFINITION('Actuator Front Cover Plate',
'Actuator Front Cover Plate',#85904,#85881);
#85904=PRODUCT_DEFINITION_FORMATION('',$,#85945);
#85940=APPLICATION_CONTEXT(
'Core Data for Automotive Mechanical Design Process');
#85941=PRODUCT_CONTEXT('part definition',#85940,'mechanical');
#85945=PRODUCT('Actuator Front Cover Plate',
'Actuator Front Cover Plate',$,(#85941));
#85964=PRESENTATION_STYLE_ASSIGNMENT((#85982));
#85982=SURFACE_STYLE_USAGE(.BOTH.,#86000);
#86000=SURFACE_SIDE_STYLE('',(#86018));
#86018=SURFACE_STYLE_FILL_AREA(#86036);
#86036=FILL_AREA_STYLE('Opaque(84,86,90)',(#86054));
#86054=FILL_AREA_STYLE_COLOUR('Opaque(84,86,90)',#86072);
#86072=COLOUR_RGB('Opaque(84,86,90)', 0.40784314, 0.44705882, 0.49803922);
ENDSEC;
END-ISO-10303-21;
